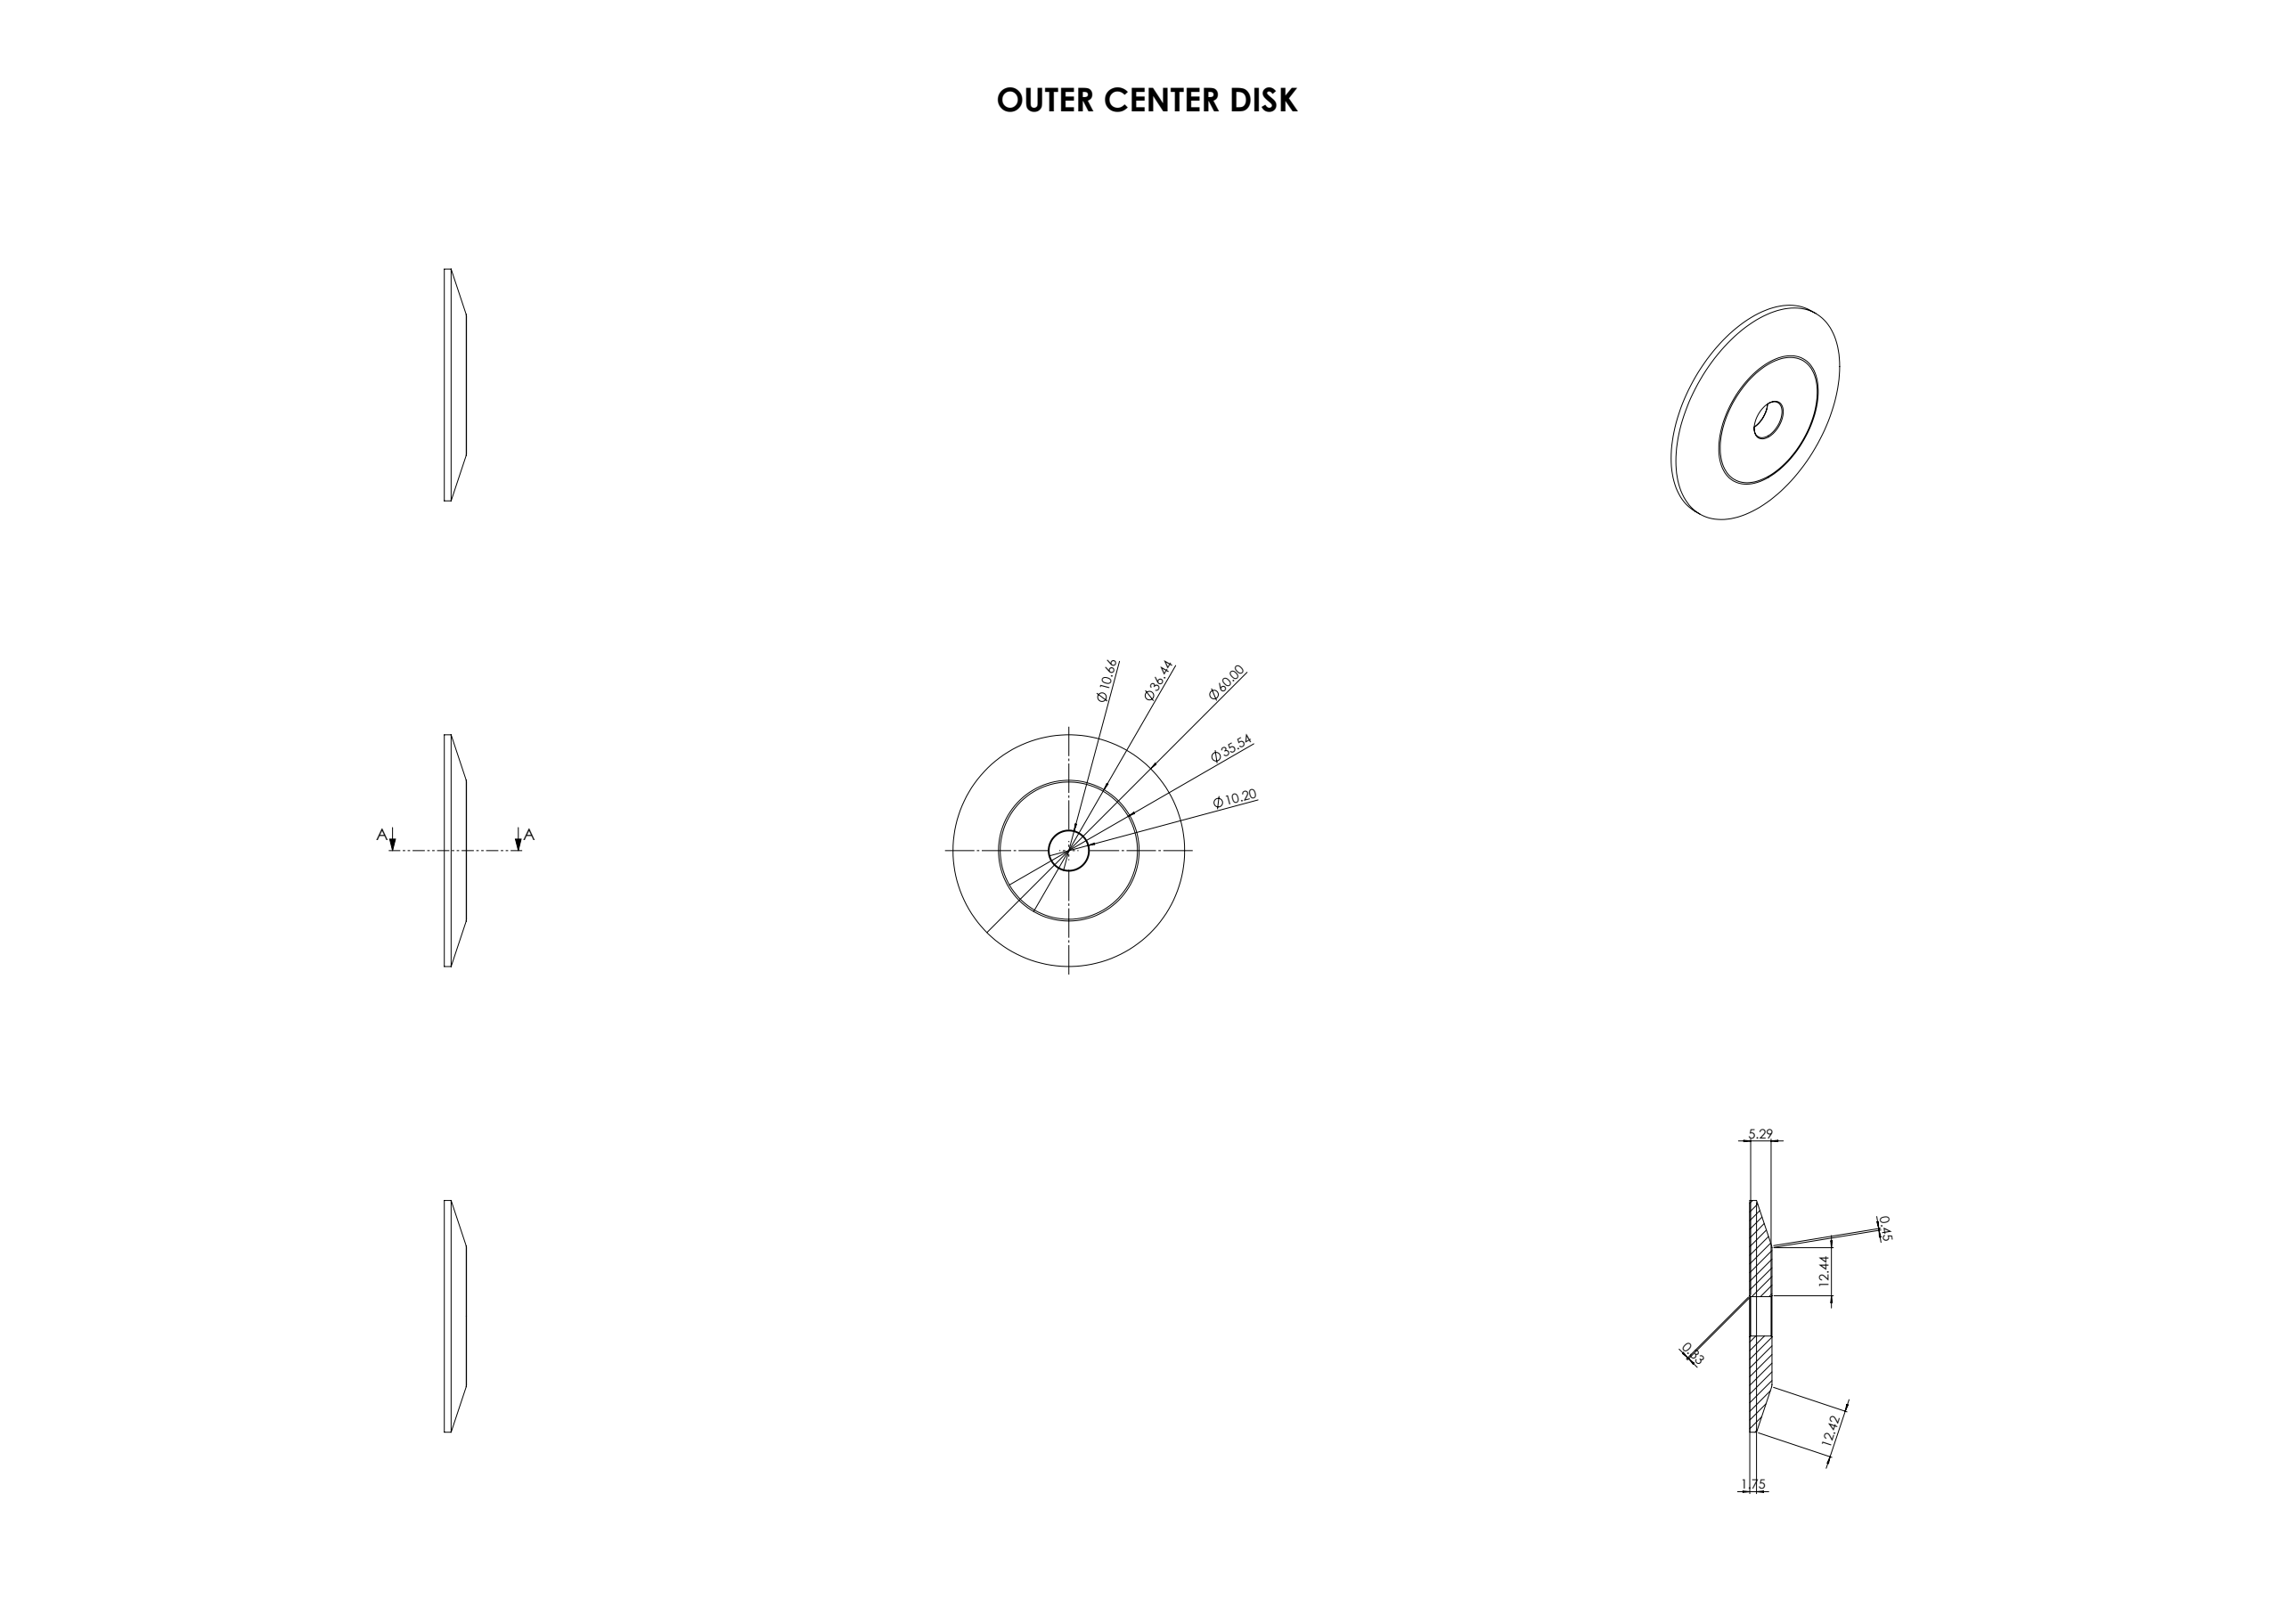
ISO-10303-21;
HEADER;
/* Generated by software containing ST-Developer
 * from STEP Tools, Inc. (www.steptools.com) 
 */

FILE_DESCRIPTION(
/* description */ (''),
/* implementation_level */ '2;1');

FILE_NAME(
/* name */ '07_Outer_Center_Disk.step',
/* time_stamp */ '2026-10-26T06:13:19-07:00',
/* author */ (''),
/* organization */ (''),
/* preprocessor_version */ 'ST-DEVELOPER v20.2',
/* originating_system */ 'Autodesk Translation Framework v15.15.0.0',
/* authorisation */ '');

FILE_SCHEMA (('AUTOMOTIVE_DESIGN { 1 0 10303 214 3 1 1 }','TECHNICAL_DATA_PACKAGING'));
ENDSEC;

DATA;
#10=MECHANICAL_DESIGN_GEOMETRIC_PRESENTATION_REPRESENTATION('',(#303),#56639);
#263=SHAPE_REPRESENTATION_RELATIONSHIP('SRR','None',#56751,#283);
#283=ADVANCED_BREP_SHAPE_REPRESENTATION('',(#323),#56625);
#303=STYLED_ITEM('',(#56908),#323);
#323=MANIFOLD_SOLID_BREP('Body1',#16955);
#508=FACE_BOUND('',#3090,.T.);
#509=FACE_BOUND('',#3095,.T.);
#591=CONICAL_SURFACE('',#17665,17.9940985792758,1.40992104959658);
#592=CONICAL_SURFACE('',#17671,24.,1.24904577239825);
#593=CONICAL_SURFACE('',#17673,5.215,0.785398163397446);
#594=CONICAL_SURFACE('',#17682,5.215,0.785398163397455);
#915=CIRCLE('',#17666,17.77);
#916=CIRCLE('',#17667,18.2181971585516);
#917=CIRCLE('',#17668,18.2181971585516);
#918=CIRCLE('',#17670,5.33);
#919=CIRCLE('',#17672,30.);
#920=CIRCLE('',#17674,5.33);
#921=CIRCLE('',#17675,5.1);
#922=CIRCLE('',#17676,5.1);
#923=CIRCLE('',#17678,5.1);
#924=CIRCLE('',#17679,5.1);
#925=CIRCLE('',#17681,30.);
#1319=CYLINDRICAL_SURFACE('',#17677,5.1);
#1320=CYLINDRICAL_SURFACE('',#17683,30.);
#2021=FACE_OUTER_BOUND('',#3088,.T.);
#2022=FACE_OUTER_BOUND('',#3089,.T.);
#2023=FACE_OUTER_BOUND('',#3091,.T.);
#2024=FACE_OUTER_BOUND('',#3092,.T.);
#2025=FACE_OUTER_BOUND('',#3093,.T.);
#2026=FACE_OUTER_BOUND('',#3094,.T.);
#2027=FACE_OUTER_BOUND('',#3096,.T.);
#2028=FACE_OUTER_BOUND('',#3097,.T.);
#3088=EDGE_LOOP('',(#11814,#11815,#11816,#11817,#11818));
#3089=EDGE_LOOP('',(#11819));
#3090=EDGE_LOOP('',(#11820));
#3091=EDGE_LOOP('',(#11821,#11822,#11823,#11824,#11825));
#3092=EDGE_LOOP('',(#11826,#11827,#11828,#11829,#11830));
#3093=EDGE_LOOP('',(#11831,#11832,#11833,#11834,#11835,#11836));
#3094=EDGE_LOOP('',(#11837));
#3095=EDGE_LOOP('',(#11838));
#3096=EDGE_LOOP('',(#11839,#11840,#11841,#11842,#11843));
#3097=EDGE_LOOP('',(#11844,#11845,#11846,#11847));
#4097=LINE('',#25089,#5051);
#4098=LINE('',#25098,#5052);
#4099=LINE('',#25104,#5053);
#4100=LINE('',#25113,#5054);
#4101=LINE('',#25118,#5055);
#4102=LINE('',#25120,#5056);
#5051=VECTOR('',#19939,17.9940985792758);
#5052=VECTOR('',#19950,24.);
#5053=VECTOR('',#19957,5.215);
#5054=VECTOR('',#19968,5.1);
#5055=VECTOR('',#19975,5.215);
#5056=VECTOR('',#19978,30.);
#7046=VERTEX_POINT('',#25086);
#7047=VERTEX_POINT('',#25088);
#7048=VERTEX_POINT('',#25090);
#7049=VERTEX_POINT('',#25094);
#7050=VERTEX_POINT('',#25097);
#7051=VERTEX_POINT('',#25101);
#7052=VERTEX_POINT('',#25103);
#7053=VERTEX_POINT('',#25105);
#7054=VERTEX_POINT('',#25109);
#7055=VERTEX_POINT('',#25110);
#7056=VERTEX_POINT('',#25115);
#8814=EDGE_CURVE('',#7046,#7046,#915,.T.);
#8815=EDGE_CURVE('',#7046,#7047,#4097,.T.);
#8816=EDGE_CURVE('',#7047,#7048,#916,.T.);
#8817=EDGE_CURVE('',#7048,#7047,#917,.T.);
#8818=EDGE_CURVE('',#7049,#7049,#918,.T.);
#8819=EDGE_CURVE('',#7048,#7050,#4098,.T.);
#8820=EDGE_CURVE('',#7050,#7050,#919,.T.);
#8821=EDGE_CURVE('',#7051,#7051,#920,.T.);
#8822=EDGE_CURVE('',#7051,#7052,#4099,.T.);
#8823=EDGE_CURVE('',#7052,#7053,#921,.T.);
#8824=EDGE_CURVE('',#7053,#7052,#922,.T.);
#8825=EDGE_CURVE('',#7054,#7055,#923,.T.);
#8826=EDGE_CURVE('',#7055,#7054,#924,.T.);
#8827=EDGE_CURVE('',#7055,#7053,#4100,.T.);
#8828=EDGE_CURVE('',#7056,#7056,#925,.T.);
#8829=EDGE_CURVE('',#7054,#7049,#4101,.T.);
#8830=EDGE_CURVE('',#7050,#7056,#4102,.T.);
#11814=ORIENTED_EDGE('',*,*,#8814,.T.);
#11815=ORIENTED_EDGE('',*,*,#8815,.T.);
#11816=ORIENTED_EDGE('',*,*,#8816,.T.);
#11817=ORIENTED_EDGE('',*,*,#8817,.T.);
#11818=ORIENTED_EDGE('',*,*,#8815,.F.);
#11819=ORIENTED_EDGE('',*,*,#8814,.F.);
#11820=ORIENTED_EDGE('',*,*,#8818,.F.);
#11821=ORIENTED_EDGE('',*,*,#8816,.F.);
#11822=ORIENTED_EDGE('',*,*,#8817,.F.);
#11823=ORIENTED_EDGE('',*,*,#8819,.T.);
#11824=ORIENTED_EDGE('',*,*,#8820,.T.);
#11825=ORIENTED_EDGE('',*,*,#8819,.F.);
#11826=ORIENTED_EDGE('',*,*,#8821,.T.);
#11827=ORIENTED_EDGE('',*,*,#8822,.T.);
#11828=ORIENTED_EDGE('',*,*,#8823,.T.);
#11829=ORIENTED_EDGE('',*,*,#8824,.T.);
#11830=ORIENTED_EDGE('',*,*,#8822,.F.);
#11831=ORIENTED_EDGE('',*,*,#8825,.F.);
#11832=ORIENTED_EDGE('',*,*,#8826,.F.);
#11833=ORIENTED_EDGE('',*,*,#8827,.T.);
#11834=ORIENTED_EDGE('',*,*,#8823,.F.);
#11835=ORIENTED_EDGE('',*,*,#8824,.F.);
#11836=ORIENTED_EDGE('',*,*,#8827,.F.);
#11837=ORIENTED_EDGE('',*,*,#8828,.F.);
#11838=ORIENTED_EDGE('',*,*,#8821,.F.);
#11839=ORIENTED_EDGE('',*,*,#8825,.T.);
#11840=ORIENTED_EDGE('',*,*,#8826,.T.);
#11841=ORIENTED_EDGE('',*,*,#8829,.T.);
#11842=ORIENTED_EDGE('',*,*,#8818,.T.);
#11843=ORIENTED_EDGE('',*,*,#8829,.F.);
#11844=ORIENTED_EDGE('',*,*,#8820,.F.);
#11845=ORIENTED_EDGE('',*,*,#8830,.T.);
#11846=ORIENTED_EDGE('',*,*,#8828,.T.);
#11847=ORIENTED_EDGE('',*,*,#8830,.F.);
#15781=PLANE('',#17669);
#15782=PLANE('',#17680);
#16192=ADVANCED_FACE('',(#2021),#591,.T.);
#16193=ADVANCED_FACE('',(#2022,#508),#15781,.T.);
#16194=ADVANCED_FACE('',(#2023),#592,.T.);
#16195=ADVANCED_FACE('',(#2024),#593,.F.);
#16196=ADVANCED_FACE('',(#2025),#1319,.F.);
#16197=ADVANCED_FACE('',(#2026,#509),#15782,.T.);
#16198=ADVANCED_FACE('',(#2027),#594,.F.);
#16199=ADVANCED_FACE('',(#2028),#1320,.T.);
#16955=CLOSED_SHELL('',(#16192,#16193,#16194,#16195,#16196,#16197,#16198,
#16199));
#17664=AXIS2_PLACEMENT_3D('',#25084,#19933,#19934);
#17665=AXIS2_PLACEMENT_3D('',#25085,#19935,#19936);
#17666=AXIS2_PLACEMENT_3D('',#25087,#19937,#19938);
#17667=AXIS2_PLACEMENT_3D('',#25091,#19940,#19941);
#17668=AXIS2_PLACEMENT_3D('',#25092,#19942,#19943);
#17669=AXIS2_PLACEMENT_3D('',#25093,#19944,#19945);
#17670=AXIS2_PLACEMENT_3D('',#25095,#19946,#19947);
#17671=AXIS2_PLACEMENT_3D('',#25096,#19948,#19949);
#17672=AXIS2_PLACEMENT_3D('',#25099,#19951,#19952);
#17673=AXIS2_PLACEMENT_3D('',#25100,#19953,#19954);
#17674=AXIS2_PLACEMENT_3D('',#25102,#19955,#19956);
#17675=AXIS2_PLACEMENT_3D('',#25106,#19958,#19959);
#17676=AXIS2_PLACEMENT_3D('',#25107,#19960,#19961);
#17677=AXIS2_PLACEMENT_3D('',#25108,#19962,#19963);
#17678=AXIS2_PLACEMENT_3D('',#25111,#19964,#19965);
#17679=AXIS2_PLACEMENT_3D('',#25112,#19966,#19967);
#17680=AXIS2_PLACEMENT_3D('',#25114,#19969,#19970);
#17681=AXIS2_PLACEMENT_3D('',#25116,#19971,#19972);
#17682=AXIS2_PLACEMENT_3D('',#25117,#19973,#19974);
#17683=AXIS2_PLACEMENT_3D('',#25119,#19976,#19977);
#19933=DIRECTION('axis',(0.,0.,1.));
#19934=DIRECTION('refdir',(1.,0.,0.));
#19935=DIRECTION('center_axis',(-1.,0.,-1.53376356854657E-14));
#19936=DIRECTION('ref_axis',(0.,-1.,-3.09974638881766E-17));
#19937=DIRECTION('center_axis',(-1.,0.,0.));
#19938=DIRECTION('ref_axis',(0.,-1.,0.));
#19939=DIRECTION('',(-0.16018224300696,0.987087457637498,-2.30533632915147E-15));
#19940=DIRECTION('center_axis',(1.,0.,0.));
#19941=DIRECTION('ref_axis',(0.,-1.,-6.12323399573677E-17));
#19942=DIRECTION('center_axis',(1.,0.,0.));
#19943=DIRECTION('ref_axis',(0.,-1.,-6.12323399573677E-17));
#19944=DIRECTION('center_axis',(1.,0.,0.));
#19945=DIRECTION('ref_axis',(0.,0.,-1.));
#19946=DIRECTION('center_axis',(1.,0.,0.));
#19947=DIRECTION('ref_axis',(0.,-1.,0.));
#19948=DIRECTION('center_axis',(-1.,0.,0.));
#19949=DIRECTION('ref_axis',(0.,1.,0.));
#19950=DIRECTION('',(-0.316227766016838,-0.948683298050514,-1.16180196436212E-16));
#19951=DIRECTION('center_axis',(1.,0.,0.));
#19952=DIRECTION('ref_axis',(0.,0.,-1.));
#19953=DIRECTION('center_axis',(-1.,0.,0.));
#19954=DIRECTION('ref_axis',(0.,-1.,0.));
#19955=DIRECTION('center_axis',(-1.,0.,0.));
#19956=DIRECTION('ref_axis',(0.,-1.,0.));
#19957=DIRECTION('',(0.707106781186549,-0.707106781186546,8.65956056235491E-17));
#19958=DIRECTION('center_axis',(1.,0.,0.));
#19959=DIRECTION('ref_axis',(0.,-1.,0.));
#19960=DIRECTION('center_axis',(1.,0.,0.));
#19961=DIRECTION('ref_axis',(0.,-1.,0.));
#19962=DIRECTION('center_axis',(1.,0.,0.));
#19963=DIRECTION('ref_axis',(0.,1.,0.));
#19964=DIRECTION('center_axis',(-1.,0.,0.));
#19965=DIRECTION('ref_axis',(0.,-1.,0.));
#19966=DIRECTION('center_axis',(-1.,0.,0.));
#19967=DIRECTION('ref_axis',(0.,-1.,0.));
#19968=DIRECTION('',(-1.,0.,0.));
#19969=DIRECTION('center_axis',(-1.,0.,0.));
#19970=DIRECTION('ref_axis',(0.,0.,1.));
#19971=DIRECTION('center_axis',(1.,0.,0.));
#19972=DIRECTION('ref_axis',(0.,0.,-1.));
#19973=DIRECTION('center_axis',(1.,0.,0.));
#19974=DIRECTION('ref_axis',(0.,-1.,0.));
#19975=DIRECTION('',(0.707106781186542,0.707106781186553,-8.659560562355E-17));
#19976=DIRECTION('center_axis',(1.,0.,0.));
#19977=DIRECTION('ref_axis',(0.,1.,0.));
#19978=DIRECTION('',(-1.,0.,0.));
#25084=CARTESIAN_POINT('',(0.,0.,0.));
#25085=CARTESIAN_POINT('Origin',(43.9636338069081,0.,-5.57771420911391E-16));
#25086=CARTESIAN_POINT('',(44.,17.77,-2.17619736208484E-15));
#25087=CARTESIAN_POINT('Origin',(44.,0.,0.));
#25088=CARTESIAN_POINT('',(43.9272676138161,18.2181971585516,2.23108568364556E-15));
#25089=CARTESIAN_POINT('',(43.9636338069081,17.9940985792758,2.2036415228652E-15));
#25090=CARTESIAN_POINT('',(43.9272676138161,-18.2181971585516,-2.23108568364556E-15));
#25091=CARTESIAN_POINT('Origin',(43.9272676138161,0.,-1.11554284182278E-15));
#25092=CARTESIAN_POINT('Origin',(43.9272676138161,0.,-1.11554284182278E-15));
#25093=CARTESIAN_POINT('Origin',(44.,5.1,0.));
#25094=CARTESIAN_POINT('',(44.,5.33,6.52736743945539E-16));
#25095=CARTESIAN_POINT('Origin',(44.,0.,0.));
#25096=CARTESIAN_POINT('Origin',(42.,0.,0.));
#25097=CARTESIAN_POINT('',(40.,-30.,-3.67394039744206E-15));
#25098=CARTESIAN_POINT('',(42.,-24.,-2.93915231795365E-15));
#25099=CARTESIAN_POINT('Origin',(40.,0.,0.));
#25100=CARTESIAN_POINT('Origin',(38.365,0.,0.));
#25101=CARTESIAN_POINT('',(38.25,5.33,-6.52736743945539E-16));
#25102=CARTESIAN_POINT('Origin',(38.25,0.,0.));
#25103=CARTESIAN_POINT('',(38.48,5.1,6.2456986756515E-16));
#25104=CARTESIAN_POINT('',(38.365,5.215,-6.38653305755345E-16));
#25105=CARTESIAN_POINT('',(38.48,-5.1,-6.2456986756515E-16));
#25106=CARTESIAN_POINT('Origin',(38.48,0.,0.));
#25107=CARTESIAN_POINT('Origin',(38.48,0.,0.));
#25108=CARTESIAN_POINT('Origin',(41.125,0.,0.));
#25109=CARTESIAN_POINT('',(43.77,5.1,-6.2456986756515E-16));
#25110=CARTESIAN_POINT('',(43.77,-5.1,-6.2456986756515E-16));
#25111=CARTESIAN_POINT('Origin',(43.77,0.,0.));
#25112=CARTESIAN_POINT('Origin',(43.77,0.,0.));
#25113=CARTESIAN_POINT('',(41.125,-5.1,-6.2456986756515E-16));
#25114=CARTESIAN_POINT('Origin',(38.25,30.,0.));
#25115=CARTESIAN_POINT('',(38.25,-30.,-3.67394039744206E-15));
#25116=CARTESIAN_POINT('Origin',(38.25,0.,0.));
#25117=CARTESIAN_POINT('Origin',(43.885,0.,0.));
#25118=CARTESIAN_POINT('',(43.885,5.215,-6.38653305755345E-16));
#25119=CARTESIAN_POINT('Origin',(39.125,0.,0.));
#25120=CARTESIAN_POINT('',(39.125,-30.,-3.67394039744206E-15));
#56603=UNCERTAINTY_MEASURE_WITH_UNIT(LENGTH_MEASURE(0.01),#56640,
'DISTANCE_ACCURACY_VALUE',
'Maximum model space distance between geometric entities at asserted c
onnectivities');
#56617=UNCERTAINTY_MEASURE_WITH_UNIT(LENGTH_MEASURE(0.01),#56640,
'DISTANCE_ACCURACY_VALUE',
'Maximum model space distance between geometric entities at asserted c
onnectivities');
#56625=(
GEOMETRIC_REPRESENTATION_CONTEXT(3)
GLOBAL_UNCERTAINTY_ASSIGNED_CONTEXT((#56603))
GLOBAL_UNIT_ASSIGNED_CONTEXT((#56640,#56642,#56643))
REPRESENTATION_CONTEXT('','3D')
);
#56639=(
GEOMETRIC_REPRESENTATION_CONTEXT(3)
GLOBAL_UNCERTAINTY_ASSIGNED_CONTEXT((#56617))
GLOBAL_UNIT_ASSIGNED_CONTEXT((#56640,#56642,#56643))
REPRESENTATION_CONTEXT('','3D')
);
#56640=(
LENGTH_UNIT()
NAMED_UNIT(*)
SI_UNIT(.MILLI.,.METRE.)
);
#56642=(
NAMED_UNIT(*)
PLANE_ANGLE_UNIT()
SI_UNIT($,.RADIAN.)
);
#56643=(
NAMED_UNIT(*)
SI_UNIT($,.STERADIAN.)
SOLID_ANGLE_UNIT()
);
#56651=SHAPE_DEFINITION_REPRESENTATION(#56672,#56751);
#56672=PRODUCT_DEFINITION_SHAPE('',$,#56773);
#56751=SHAPE_REPRESENTATION('',(#17664),#56625);
#56765=PRODUCT_DEFINITION_CONTEXT('part definition',#56830,'design');
#56773=PRODUCT_DEFINITION('2026-10-26-00-02-42-500',
'07_Outer_Center_Disk',#56794,#56765);
#56794=PRODUCT_DEFINITION_FORMATION('',$,#56839);
#56830=APPLICATION_CONTEXT(
'Core Data for Automotive Mechanical Design Process');
#56831=PRODUCT_CONTEXT('part definition',#56830,'mechanical');
#56839=PRODUCT('2026-10-26-00-02-42-500','07_Outer_Center_Disk',$,(#56831));
#56902=COLOUR_RGB('Sky Blue',0.24,0.69,0.87);
#56903=FILL_AREA_STYLE_COLOUR('',#56902);
#56904=FILL_AREA_STYLE('',(#56903));
#56905=SURFACE_STYLE_FILL_AREA(#56904);
#56906=SURFACE_SIDE_STYLE('',(#56905));
#56907=SURFACE_STYLE_USAGE(.BOTH.,#56906);
#56908=PRESENTATION_STYLE_ASSIGNMENT((#56907));
ENDSEC;
END-ISO-10303-21;
